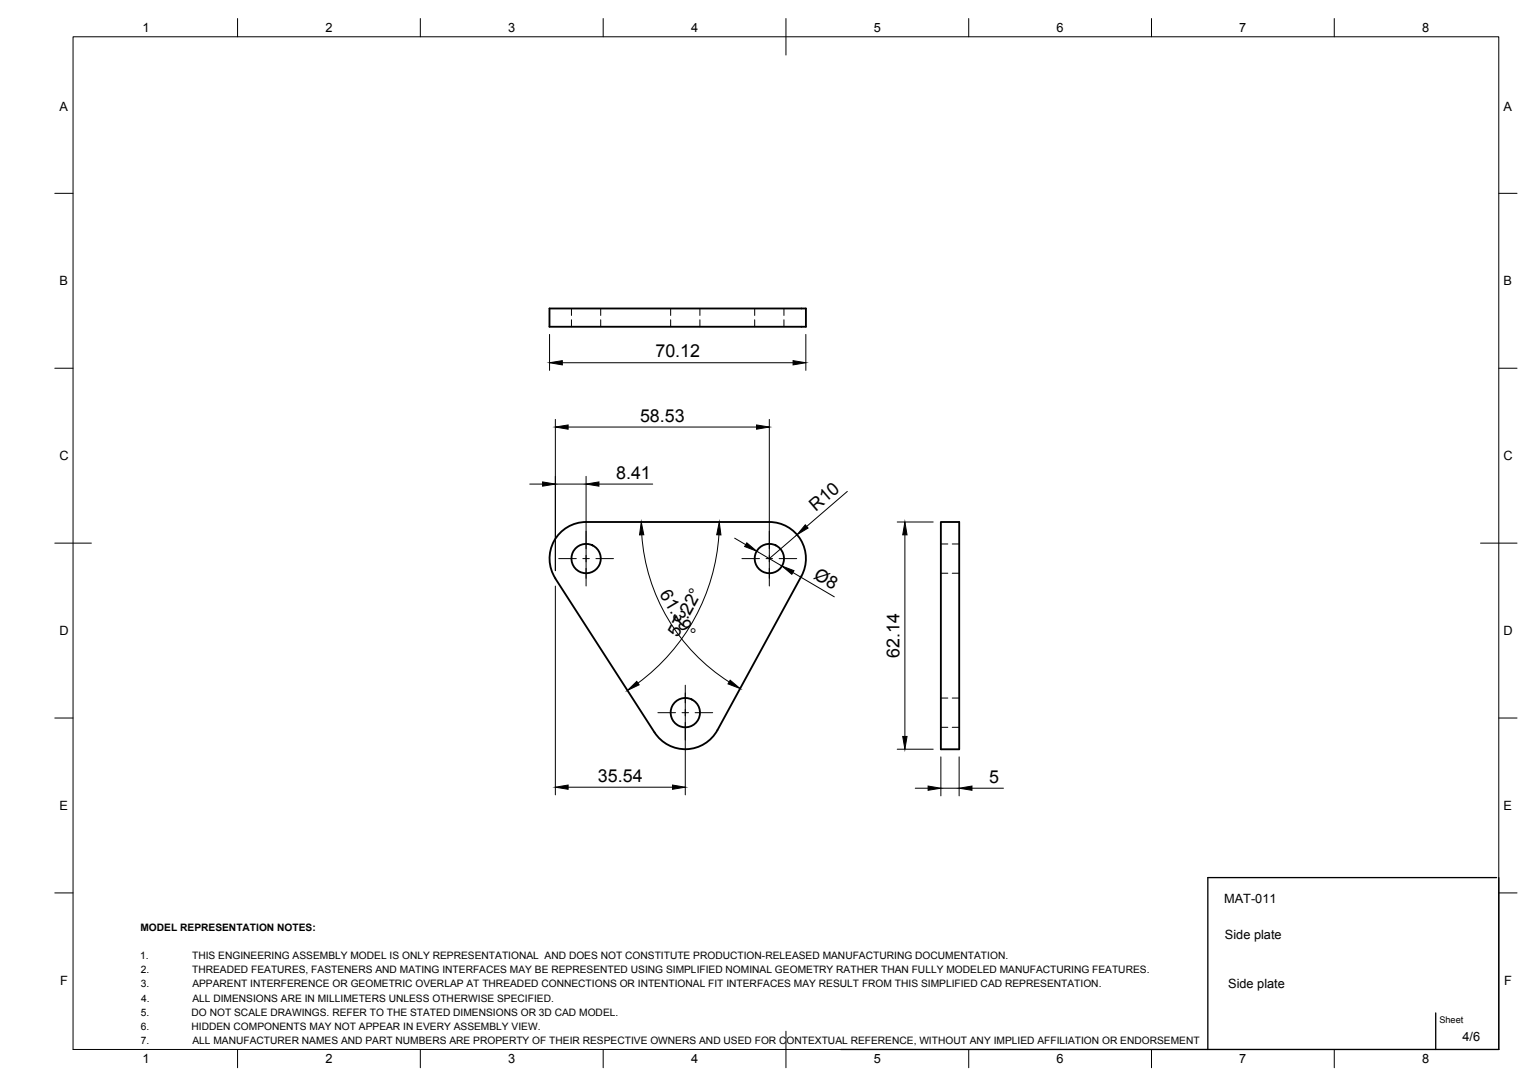
ISO-10303-21;
HEADER;
/* Generated by software containing ST-Developer
 * from STEP Tools, Inc. (www.steptools.com) 
 */

FILE_DESCRIPTION(
/* description */ ('STEP AP214'),
/* implementation_level */ '2;1');

FILE_NAME(
/* name */ 'Side Plate.step',
/* time_stamp */ '2026-11-14T05:56:09-08:00',
/* author */ (''),
/* organization */ (''),
/* preprocessor_version */ 'ST-DEVELOPER v20.2',
/* originating_system */ 'Autodesk Translation Framework v15.17.0.0',
/* authorisation */ '');

FILE_SCHEMA (('AUTOMOTIVE_DESIGN { 1 0 10303 214 3 1 1 }'));
ENDSEC;

DATA;
#10=MECHANICAL_DESIGN_GEOMETRIC_PRESENTATION_REPRESENTATION('',(#105),#3207);
#93=SHAPE_REPRESENTATION_RELATIONSHIP('SRR','None',#3245,#99);
#99=ADVANCED_BREP_SHAPE_REPRESENTATION('',(#111),#3204);
#105=STYLED_ITEM('',(#3281),#111);
#111=MANIFOLD_SOLID_BREP('Body1',#1283);
#133=PLANE('',#1429);
#134=PLANE('',#1432);
#135=PLANE('',#1435);
#136=PLANE('',#1437);
#137=PLANE('',#1439);
#187=LINE('',#2105,#254);
#188=LINE('',#2111,#255);
#189=LINE('',#2117,#256);
#190=LINE('',#2124,#257);
#191=LINE('',#2127,#258);
#192=LINE('',#2130,#259);
#193=LINE('',#2134,#260);
#194=LINE('',#2137,#261);
#195=LINE('',#2140,#262);
#196=LINE('',#2144,#263);
#197=LINE('',#2147,#264);
#198=LINE('',#2149,#265);
#199=LINE('',#2151,#266);
#200=LINE('',#2153,#267);
#201=LINE('',#2155,#268);
#254=VECTOR('',#1685,4.);
#255=VECTOR('',#1692,4.);
#256=VECTOR('',#1699,4.);
#257=VECTOR('',#1706,1000.);
#258=VECTOR('',#1709,1000.);
#259=VECTOR('',#1712,1000.);
#260=VECTOR('',#1715,1000.);
#261=VECTOR('',#1718,1000.);
#262=VECTOR('',#1721,1000.);
#263=VECTOR('',#1724,1000.);
#264=VECTOR('',#1727,1000.);
#265=VECTOR('',#1730,1000.);
#266=VECTOR('',#1733,1000.);
#267=VECTOR('',#1736,1000.);
#268=VECTOR('',#1739,1000.);
#293=CYLINDRICAL_SURFACE('',#1417,4.);
#294=CYLINDRICAL_SURFACE('',#1420,4.);
#295=CYLINDRICAL_SURFACE('',#1423,4.);
#296=CYLINDRICAL_SURFACE('',#1426,10.);
#297=CYLINDRICAL_SURFACE('',#1436,9.99999951505478);
#298=CYLINDRICAL_SURFACE('',#1438,10.);
#314=FACE_BOUND('',#463,.T.);
#315=FACE_BOUND('',#464,.T.);
#316=FACE_BOUND('',#465,.T.);
#317=FACE_BOUND('',#467,.T.);
#318=FACE_BOUND('',#468,.T.);
#319=FACE_BOUND('',#469,.T.);
#377=FACE_OUTER_BOUND('',#458,.T.);
#378=FACE_OUTER_BOUND('',#459,.T.);
#379=FACE_OUTER_BOUND('',#460,.T.);
#380=FACE_OUTER_BOUND('',#461,.T.);
#381=FACE_OUTER_BOUND('',#462,.T.);
#382=FACE_OUTER_BOUND('',#466,.T.);
#383=FACE_OUTER_BOUND('',#470,.T.);
#384=FACE_OUTER_BOUND('',#471,.T.);
#385=FACE_OUTER_BOUND('',#472,.T.);
#386=FACE_OUTER_BOUND('',#473,.T.);
#387=FACE_OUTER_BOUND('',#474,.T.);
#458=EDGE_LOOP('',(#991,#992,#993,#994));
#459=EDGE_LOOP('',(#995,#996,#997,#998));
#460=EDGE_LOOP('',(#999,#1000,#1001,#1002));
#461=EDGE_LOOP('',(#1003,#1004,#1005,#1006));
#462=EDGE_LOOP('',(#1007,#1008,#1009,#1010,#1011,#1012));
#463=EDGE_LOOP('',(#1013));
#464=EDGE_LOOP('',(#1014));
#465=EDGE_LOOP('',(#1015));
#466=EDGE_LOOP('',(#1016,#1017,#1018,#1019,#1020,#1021));
#467=EDGE_LOOP('',(#1022));
#468=EDGE_LOOP('',(#1023));
#469=EDGE_LOOP('',(#1024));
#470=EDGE_LOOP('',(#1025,#1026,#1027,#1028));
#471=EDGE_LOOP('',(#1029,#1030,#1031,#1032));
#472=EDGE_LOOP('',(#1033,#1034,#1035,#1036));
#473=EDGE_LOOP('',(#1037,#1038,#1039,#1040));
#474=EDGE_LOOP('',(#1041,#1042,#1043,#1044));
#545=CIRCLE('',#1418,4.);
#546=CIRCLE('',#1419,4.);
#547=CIRCLE('',#1421,4.);
#548=CIRCLE('',#1422,4.);
#549=CIRCLE('',#1424,4.);
#550=CIRCLE('',#1425,4.);
#551=CIRCLE('',#1427,10.);
#552=CIRCLE('',#1428,10.);
#553=CIRCLE('',#1430,9.99999951505478);
#554=CIRCLE('',#1431,10.);
#555=CIRCLE('',#1433,10.);
#556=CIRCLE('',#1434,9.99999951505478);
#627=VERTEX_POINT('',#2102);
#628=VERTEX_POINT('',#2104);
#629=VERTEX_POINT('',#2108);
#630=VERTEX_POINT('',#2110);
#631=VERTEX_POINT('',#2114);
#632=VERTEX_POINT('',#2116);
#633=VERTEX_POINT('',#2120);
#634=VERTEX_POINT('',#2121);
#635=VERTEX_POINT('',#2123);
#636=VERTEX_POINT('',#2125);
#637=VERTEX_POINT('',#2129);
#638=VERTEX_POINT('',#2131);
#639=VERTEX_POINT('',#2133);
#640=VERTEX_POINT('',#2135);
#641=VERTEX_POINT('',#2139);
#642=VERTEX_POINT('',#2141);
#643=VERTEX_POINT('',#2143);
#644=VERTEX_POINT('',#2145);
#759=EDGE_CURVE('',#627,#627,#545,.T.);
#760=EDGE_CURVE('',#627,#628,#187,.T.);
#761=EDGE_CURVE('',#628,#628,#546,.T.);
#762=EDGE_CURVE('',#629,#629,#547,.T.);
#763=EDGE_CURVE('',#629,#630,#188,.T.);
#764=EDGE_CURVE('',#630,#630,#548,.T.);
#765=EDGE_CURVE('',#631,#631,#549,.T.);
#766=EDGE_CURVE('',#631,#632,#189,.T.);
#767=EDGE_CURVE('',#632,#632,#550,.T.);
#768=EDGE_CURVE('',#633,#634,#551,.T.);
#769=EDGE_CURVE('',#633,#635,#190,.T.);
#770=EDGE_CURVE('',#635,#636,#552,.T.);
#771=EDGE_CURVE('',#634,#636,#191,.T.);
#772=EDGE_CURVE('',#634,#637,#192,.T.);
#773=EDGE_CURVE('',#637,#638,#553,.T.);
#774=EDGE_CURVE('',#638,#639,#193,.T.);
#775=EDGE_CURVE('',#639,#640,#554,.T.);
#776=EDGE_CURVE('',#640,#633,#194,.T.);
#777=EDGE_CURVE('',#641,#635,#195,.T.);
#778=EDGE_CURVE('',#642,#641,#555,.T.);
#779=EDGE_CURVE('',#643,#642,#196,.T.);
#780=EDGE_CURVE('',#644,#643,#556,.T.);
#781=EDGE_CURVE('',#636,#644,#197,.T.);
#782=EDGE_CURVE('',#637,#644,#198,.T.);
#783=EDGE_CURVE('',#638,#643,#199,.T.);
#784=EDGE_CURVE('',#639,#642,#200,.T.);
#785=EDGE_CURVE('',#640,#641,#201,.T.);
#991=ORIENTED_EDGE('',*,*,#759,.T.);
#992=ORIENTED_EDGE('',*,*,#760,.T.);
#993=ORIENTED_EDGE('',*,*,#761,.F.);
#994=ORIENTED_EDGE('',*,*,#760,.F.);
#995=ORIENTED_EDGE('',*,*,#762,.T.);
#996=ORIENTED_EDGE('',*,*,#763,.T.);
#997=ORIENTED_EDGE('',*,*,#764,.F.);
#998=ORIENTED_EDGE('',*,*,#763,.F.);
#999=ORIENTED_EDGE('',*,*,#765,.T.);
#1000=ORIENTED_EDGE('',*,*,#766,.T.);
#1001=ORIENTED_EDGE('',*,*,#767,.F.);
#1002=ORIENTED_EDGE('',*,*,#766,.F.);
#1003=ORIENTED_EDGE('',*,*,#768,.F.);
#1004=ORIENTED_EDGE('',*,*,#769,.T.);
#1005=ORIENTED_EDGE('',*,*,#770,.T.);
#1006=ORIENTED_EDGE('',*,*,#771,.F.);
#1007=ORIENTED_EDGE('',*,*,#768,.T.);
#1008=ORIENTED_EDGE('',*,*,#772,.T.);
#1009=ORIENTED_EDGE('',*,*,#773,.T.);
#1010=ORIENTED_EDGE('',*,*,#774,.T.);
#1011=ORIENTED_EDGE('',*,*,#775,.T.);
#1012=ORIENTED_EDGE('',*,*,#776,.T.);
#1013=ORIENTED_EDGE('',*,*,#765,.F.);
#1014=ORIENTED_EDGE('',*,*,#759,.F.);
#1015=ORIENTED_EDGE('',*,*,#762,.F.);
#1016=ORIENTED_EDGE('',*,*,#770,.F.);
#1017=ORIENTED_EDGE('',*,*,#777,.F.);
#1018=ORIENTED_EDGE('',*,*,#778,.F.);
#1019=ORIENTED_EDGE('',*,*,#779,.F.);
#1020=ORIENTED_EDGE('',*,*,#780,.F.);
#1021=ORIENTED_EDGE('',*,*,#781,.F.);
#1022=ORIENTED_EDGE('',*,*,#767,.T.);
#1023=ORIENTED_EDGE('',*,*,#761,.T.);
#1024=ORIENTED_EDGE('',*,*,#764,.T.);
#1025=ORIENTED_EDGE('',*,*,#781,.T.);
#1026=ORIENTED_EDGE('',*,*,#782,.F.);
#1027=ORIENTED_EDGE('',*,*,#772,.F.);
#1028=ORIENTED_EDGE('',*,*,#771,.T.);
#1029=ORIENTED_EDGE('',*,*,#780,.T.);
#1030=ORIENTED_EDGE('',*,*,#783,.F.);
#1031=ORIENTED_EDGE('',*,*,#773,.F.);
#1032=ORIENTED_EDGE('',*,*,#782,.T.);
#1033=ORIENTED_EDGE('',*,*,#779,.T.);
#1034=ORIENTED_EDGE('',*,*,#784,.F.);
#1035=ORIENTED_EDGE('',*,*,#774,.F.);
#1036=ORIENTED_EDGE('',*,*,#783,.T.);
#1037=ORIENTED_EDGE('',*,*,#778,.T.);
#1038=ORIENTED_EDGE('',*,*,#785,.F.);
#1039=ORIENTED_EDGE('',*,*,#775,.F.);
#1040=ORIENTED_EDGE('',*,*,#784,.T.);
#1041=ORIENTED_EDGE('',*,*,#777,.T.);
#1042=ORIENTED_EDGE('',*,*,#769,.F.);
#1043=ORIENTED_EDGE('',*,*,#776,.F.);
#1044=ORIENTED_EDGE('',*,*,#785,.T.);
#1235=ADVANCED_FACE('',(#377),#293,.F.);
#1236=ADVANCED_FACE('',(#378),#294,.F.);
#1237=ADVANCED_FACE('',(#379),#295,.F.);
#1238=ADVANCED_FACE('',(#380),#296,.T.);
#1239=ADVANCED_FACE('',(#381,#314,#315,#316),#133,.T.);
#1240=ADVANCED_FACE('',(#382,#317,#318,#319),#134,.F.);
#1241=ADVANCED_FACE('',(#383),#135,.F.);
#1242=ADVANCED_FACE('',(#384),#297,.T.);
#1243=ADVANCED_FACE('',(#385),#136,.F.);
#1244=ADVANCED_FACE('',(#386),#298,.T.);
#1245=ADVANCED_FACE('',(#387),#137,.F.);
#1283=CLOSED_SHELL('',(#1235,#1236,#1237,#1238,#1239,#1240,#1241,#1242,
#1243,#1244,#1245));
#1416=AXIS2_PLACEMENT_3D('',#2100,#1679,#1680);
#1417=AXIS2_PLACEMENT_3D('',#2101,#1681,#1682);
#1418=AXIS2_PLACEMENT_3D('',#2103,#1683,#1684);
#1419=AXIS2_PLACEMENT_3D('',#2106,#1686,#1687);
#1420=AXIS2_PLACEMENT_3D('',#2107,#1688,#1689);
#1421=AXIS2_PLACEMENT_3D('',#2109,#1690,#1691);
#1422=AXIS2_PLACEMENT_3D('',#2112,#1693,#1694);
#1423=AXIS2_PLACEMENT_3D('',#2113,#1695,#1696);
#1424=AXIS2_PLACEMENT_3D('',#2115,#1697,#1698);
#1425=AXIS2_PLACEMENT_3D('',#2118,#1700,#1701);
#1426=AXIS2_PLACEMENT_3D('',#2119,#1702,#1703);
#1427=AXIS2_PLACEMENT_3D('',#2122,#1704,#1705);
#1428=AXIS2_PLACEMENT_3D('',#2126,#1707,#1708);
#1429=AXIS2_PLACEMENT_3D('',#2128,#1710,#1711);
#1430=AXIS2_PLACEMENT_3D('',#2132,#1713,#1714);
#1431=AXIS2_PLACEMENT_3D('',#2136,#1716,#1717);
#1432=AXIS2_PLACEMENT_3D('',#2138,#1719,#1720);
#1433=AXIS2_PLACEMENT_3D('',#2142,#1722,#1723);
#1434=AXIS2_PLACEMENT_3D('',#2146,#1725,#1726);
#1435=AXIS2_PLACEMENT_3D('',#2148,#1728,#1729);
#1436=AXIS2_PLACEMENT_3D('',#2150,#1731,#1732);
#1437=AXIS2_PLACEMENT_3D('',#2152,#1734,#1735);
#1438=AXIS2_PLACEMENT_3D('',#2154,#1737,#1738);
#1439=AXIS2_PLACEMENT_3D('',#2156,#1740,#1741);
#1679=DIRECTION('axis',(0.,0.,1.));
#1680=DIRECTION('refdir',(1.,0.,0.));
#1681=DIRECTION('center_axis',(0.,0.,-1.));
#1682=DIRECTION('ref_axis',(-1.,0.,0.));
#1683=DIRECTION('center_axis',(0.,0.,1.));
#1684=DIRECTION('ref_axis',(1.,0.,0.));
#1685=DIRECTION('',(0.,0.,-1.));
#1686=DIRECTION('center_axis',(0.,0.,1.));
#1687=DIRECTION('ref_axis',(1.,0.,0.));
#1688=DIRECTION('center_axis',(0.,0.,-1.));
#1689=DIRECTION('ref_axis',(-1.,0.,0.));
#1690=DIRECTION('center_axis',(0.,0.,1.));
#1691=DIRECTION('ref_axis',(1.,0.,0.));
#1692=DIRECTION('',(0.,0.,-1.));
#1693=DIRECTION('center_axis',(0.,0.,1.));
#1694=DIRECTION('ref_axis',(1.,0.,0.));
#1695=DIRECTION('center_axis',(0.,0.,-1.));
#1696=DIRECTION('ref_axis',(-1.,0.,0.));
#1697=DIRECTION('center_axis',(0.,0.,1.));
#1698=DIRECTION('ref_axis',(1.,0.,0.));
#1699=DIRECTION('',(0.,0.,-1.));
#1700=DIRECTION('center_axis',(0.,0.,1.));
#1701=DIRECTION('ref_axis',(1.,0.,0.));
#1702=DIRECTION('center_axis',(0.,0.,-1.));
#1703=DIRECTION('ref_axis',(-1.,0.,0.));
#1704=DIRECTION('center_axis',(0.,0.,1.));
#1705=DIRECTION('ref_axis',(1.,0.,0.));
#1706=DIRECTION('',(0.,0.,-1.));
#1707=DIRECTION('center_axis',(0.,0.,1.));
#1708=DIRECTION('ref_axis',(1.,0.,0.));
#1709=DIRECTION('',(0.,0.,-1.));
#1710=DIRECTION('center_axis',(0.,0.,1.));
#1711=DIRECTION('ref_axis',(1.,0.,0.));
#1712=DIRECTION('',(0.478852136424395,-0.87789556978139,0.));
#1713=DIRECTION('center_axis',(0.,0.,1.));
#1714=DIRECTION('ref_axis',(1.,0.,0.));
#1715=DIRECTION('',(0.478852136424396,0.87789556978139,0.));
#1716=DIRECTION('center_axis',(0.,0.,1.));
#1717=DIRECTION('ref_axis',(1.,0.,0.));
#1718=DIRECTION('',(-1.,-1.44560289664734E-16,0.));
#1719=DIRECTION('center_axis',(0.,0.,1.));
#1720=DIRECTION('ref_axis',(1.,0.,0.));
#1721=DIRECTION('',(-1.,-1.44560289664734E-16,0.));
#1722=DIRECTION('center_axis',(0.,0.,1.));
#1723=DIRECTION('ref_axis',(1.,0.,0.));
#1724=DIRECTION('',(0.478852136424396,0.87789556978139,0.));
#1725=DIRECTION('center_axis',(0.,0.,1.));
#1726=DIRECTION('ref_axis',(1.,0.,0.));
#1727=DIRECTION('',(0.478852136424395,-0.87789556978139,0.));
#1728=DIRECTION('center_axis',(0.877895569781391,0.478852136424395,0.));
#1729=DIRECTION('ref_axis',(-0.478852136424395,0.877895569781391,0.));
#1730=DIRECTION('',(0.,0.,-1.));
#1731=DIRECTION('center_axis',(0.,0.,-1.));
#1732=DIRECTION('ref_axis',(-1.,0.,0.));
#1733=DIRECTION('',(0.,0.,-1.));
#1734=DIRECTION('center_axis',(-0.87789556978139,0.478852136424395,0.));
#1735=DIRECTION('ref_axis',(-0.478852136424395,-0.87789556978139,0.));
#1736=DIRECTION('',(0.,0.,-1.));
#1737=DIRECTION('center_axis',(0.,0.,-1.));
#1738=DIRECTION('ref_axis',(0.859898870921574,0.510464427543979,0.));
#1739=DIRECTION('',(0.,0.,-1.));
#1740=DIRECTION('center_axis',(1.44560289664734E-16,-1.,0.));
#1741=DIRECTION('ref_axis',(1.,1.44560289664734E-16,0.));
#2100=CARTESIAN_POINT('',(0.,0.,0.));
#2101=CARTESIAN_POINT('Origin',(0.,0.,5.));
#2102=CARTESIAN_POINT('',(4.,-4.89858719658941E-16,5.));
#2103=CARTESIAN_POINT('Origin',(0.,0.,5.));
#2104=CARTESIAN_POINT('',(4.,-4.89858719658941E-16,0.));
#2105=CARTESIAN_POINT('',(4.,-4.89858719658941E-16,5.));
#2106=CARTESIAN_POINT('Origin',(0.,0.,0.));
#2107=CARTESIAN_POINT('Origin',(24.,44.00000032792,5.));
#2108=CARTESIAN_POINT('',(28.,44.00000032792,5.));
#2109=CARTESIAN_POINT('Origin',(24.,44.00000032792,5.));
#2110=CARTESIAN_POINT('',(28.,44.00000032792,0.));
#2111=CARTESIAN_POINT('',(28.,44.00000032792,5.));
#2112=CARTESIAN_POINT('Origin',(24.,44.00000032792,0.));
#2113=CARTESIAN_POINT('Origin',(-24.,44.00000032792,5.));
#2114=CARTESIAN_POINT('',(-20.,44.00000032792,5.));
#2115=CARTESIAN_POINT('Origin',(-24.,44.00000032792,5.));
#2116=CARTESIAN_POINT('',(-20.,44.00000032792,0.));
#2117=CARTESIAN_POINT('',(-20.,44.00000032792,5.));
#2118=CARTESIAN_POINT('Origin',(-24.,44.00000032792,0.));
#2119=CARTESIAN_POINT('Origin',(-24.,44.00000032792,5.));
#2120=CARTESIAN_POINT('',(-24.,54.00000032792,5.));
#2121=CARTESIAN_POINT('',(-32.7789556978139,39.2114789636761,5.));
#2122=CARTESIAN_POINT('Origin',(-24.,44.00000032792,5.));
#2123=CARTESIAN_POINT('',(-24.,54.00000032792,0.));
#2124=CARTESIAN_POINT('',(-24.,54.00000032792,5.));
#2125=CARTESIAN_POINT('',(-32.7789556978139,39.2114789636761,0.));
#2126=CARTESIAN_POINT('Origin',(-24.,44.00000032792,0.));
#2127=CARTESIAN_POINT('',(-32.7789556978139,39.2114789636761,5.));
#2128=CARTESIAN_POINT('Origin',(-24.,44.00000032792,5.));
#2129=CARTESIAN_POINT('',(-8.77895527208265,-4.7885211320269,5.));
#2130=CARTESIAN_POINT('',(-32.7789556978139,39.2114789636761,5.));
#2131=CARTESIAN_POINT('',(8.77895544126431,-4.78852082186052,5.));
#2132=CARTESIAN_POINT('Origin',(0.,0.,5.));
#2133=CARTESIAN_POINT('',(32.7789556978139,39.2114789636761,5.));
#2134=CARTESIAN_POINT('',(8.77895544126431,-4.78852082186051,5.));
#2135=CARTESIAN_POINT('',(24.,54.00000032792,5.));
#2136=CARTESIAN_POINT('Origin',(24.,44.00000032792,5.));
#2137=CARTESIAN_POINT('',(24.,54.00000032792,5.));
#2138=CARTESIAN_POINT('Origin',(-24.,44.00000032792,0.));
#2139=CARTESIAN_POINT('',(24.,54.00000032792,0.));
#2140=CARTESIAN_POINT('',(24.,54.00000032792,0.));
#2141=CARTESIAN_POINT('',(32.7789556978139,39.2114789636761,0.));
#2142=CARTESIAN_POINT('Origin',(24.,44.00000032792,0.));
#2143=CARTESIAN_POINT('',(8.77895544126431,-4.78852082186052,0.));
#2144=CARTESIAN_POINT('',(8.77895544126431,-4.78852082186051,0.));
#2145=CARTESIAN_POINT('',(-8.77895527208265,-4.7885211320269,0.));
#2146=CARTESIAN_POINT('Origin',(0.,0.,0.));
#2147=CARTESIAN_POINT('',(-32.7789556978139,39.2114789636761,0.));
#2148=CARTESIAN_POINT('Origin',(-32.7789556978139,39.2114789636761,5.));
#2149=CARTESIAN_POINT('',(-8.77895527208265,-4.7885211320269,5.));
#2150=CARTESIAN_POINT('Origin',(0.,0.,5.));
#2151=CARTESIAN_POINT('',(8.77895544126431,-4.78852082186052,5.));
#2152=CARTESIAN_POINT('Origin',(8.77895544126431,-4.78852082186051,5.));
#2153=CARTESIAN_POINT('',(32.7789556978139,39.2114789636761,5.));
#2154=CARTESIAN_POINT('Origin',(24.,44.00000032792,5.));
#2155=CARTESIAN_POINT('',(24.,54.00000032792,5.));
#2156=CARTESIAN_POINT('Origin',(24.,54.00000032792,5.));
#3196=UNCERTAINTY_MEASURE_WITH_UNIT(LENGTH_MEASURE(0.01),#3208,
'DISTANCE_ACCURACY_VALUE',
'Maximum model space distance between geometric entities at asserted c
onnectivities');
#3199=UNCERTAINTY_MEASURE_WITH_UNIT(LENGTH_MEASURE(0.01),#3208,
'DISTANCE_ACCURACY_VALUE',
'Maximum model space distance between geometric entities at asserted c
onnectivities');
#3204=(
GEOMETRIC_REPRESENTATION_CONTEXT(3)
GLOBAL_UNCERTAINTY_ASSIGNED_CONTEXT((#3196))
GLOBAL_UNIT_ASSIGNED_CONTEXT((#3208,#3210,#3211))
REPRESENTATION_CONTEXT('','3D')
);
#3207=(
GEOMETRIC_REPRESENTATION_CONTEXT(3)
GLOBAL_UNCERTAINTY_ASSIGNED_CONTEXT((#3199))
GLOBAL_UNIT_ASSIGNED_CONTEXT((#3208,#3210,#3211))
REPRESENTATION_CONTEXT('','3D')
);
#3208=(
LENGTH_UNIT()
NAMED_UNIT(*)
SI_UNIT(.MILLI.,.METRE.)
);
#3210=(
NAMED_UNIT(*)
PLANE_ANGLE_UNIT()
SI_UNIT($,.RADIAN.)
);
#3211=(
NAMED_UNIT(*)
SI_UNIT($,.STERADIAN.)
SOLID_ANGLE_UNIT()
);
#3216=SHAPE_DEFINITION_REPRESENTATION(#3223,#3245);
#3223=PRODUCT_DEFINITION_SHAPE('',$,#3253);
#3245=SHAPE_REPRESENTATION('',(#1416),#3204);
#3248=PRODUCT_DEFINITION_CONTEXT('part definition',#3271,'design');
#3253=PRODUCT_DEFINITION('Side plate','Side Plate',#3260,#3248);
#3260=PRODUCT_DEFINITION_FORMATION('',$,#3277);
#3271=APPLICATION_CONTEXT(
'Core Data for Automotive Mechanical Design Process');
#3272=PRODUCT_CONTEXT('part definition',#3271,'mechanical');
#3277=PRODUCT('Side plate','Side Plate','Side plate',(#3272));
#3281=PRESENTATION_STYLE_ASSIGNMENT((#3285));
#3285=SURFACE_STYLE_USAGE(.BOTH.,#3289);
#3289=SURFACE_SIDE_STYLE('',(#3293));
#3293=SURFACE_STYLE_FILL_AREA(#3297);
#3297=FILL_AREA_STYLE('Opaque(97,158,199)',(#3301));
#3301=FILL_AREA_STYLE_COLOUR('Opaque(97,158,199)',#3305);
#3305=COLOUR_RGB('Opaque(97,158,199)',0.380392156862745,0.619607843137255,
0.780392156862745);
ENDSEC;
END-ISO-10303-21;
